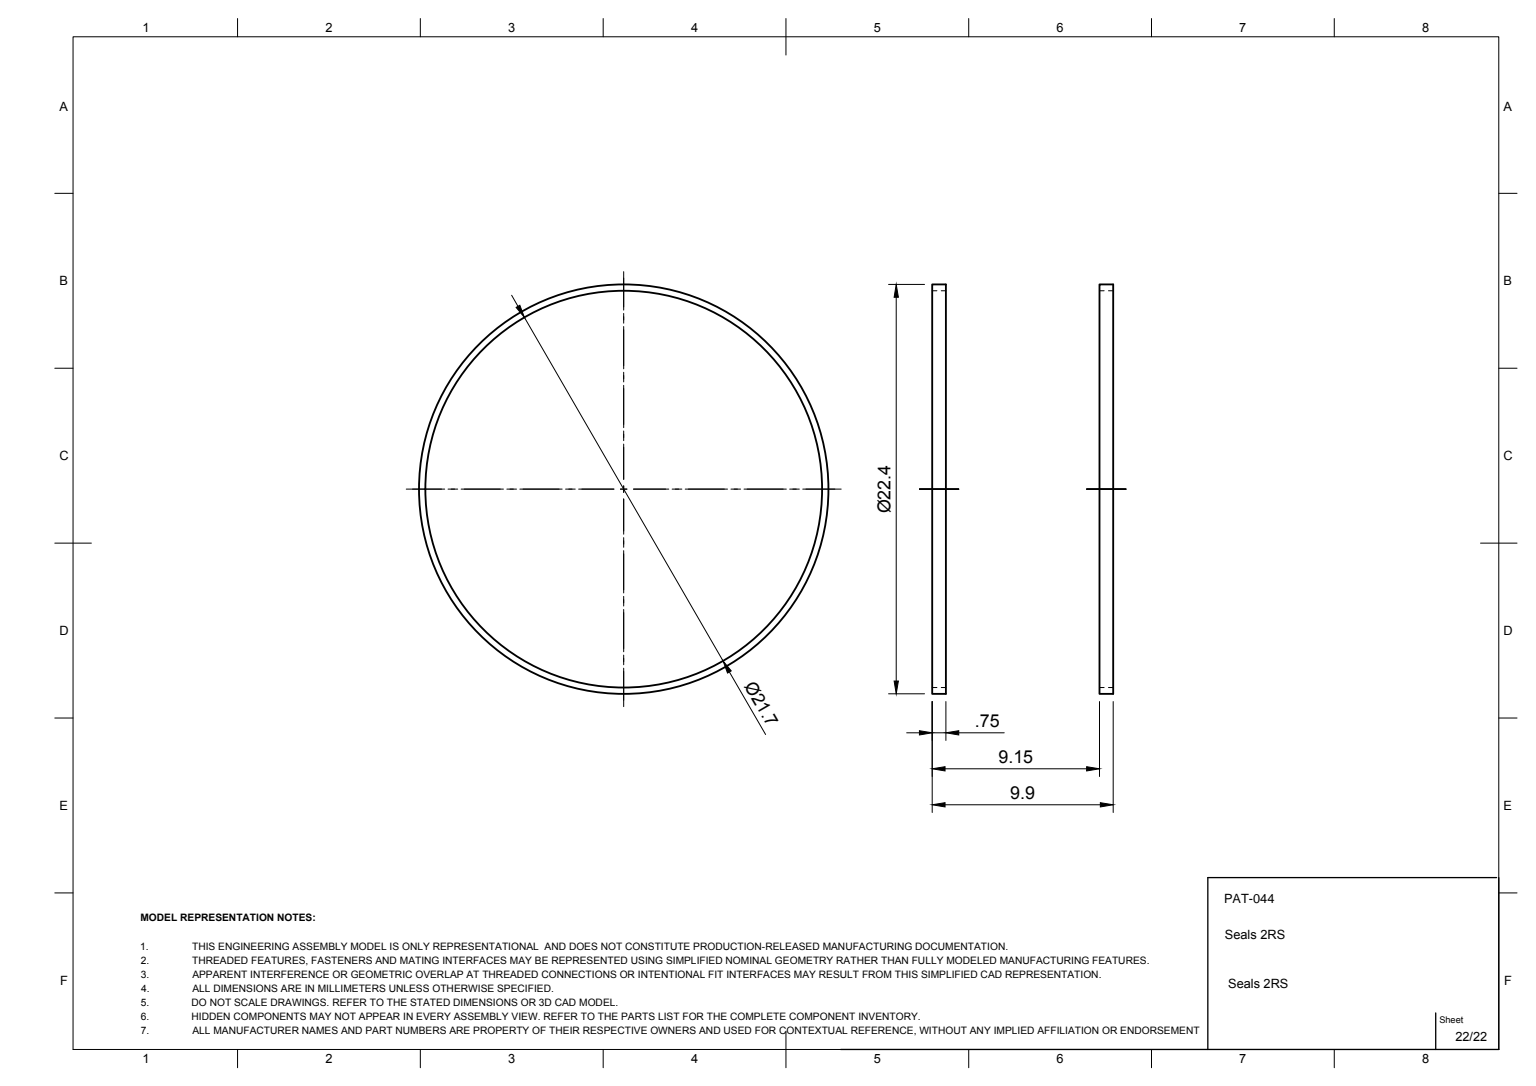
ISO-10303-21;
HEADER;
/* Generated by software containing ST-Developer
 * from STEP Tools, Inc. (www.steptools.com) 
 */

FILE_DESCRIPTION(
/* description */ ('Four-wheel beam trolley'),
/* implementation_level */ '2;1');

FILE_NAME(
/* name */ 'Seals 2RS.step',
/* time_stamp */ '2026-10-29T16:22:06-07:00',
/* author */ (''),
/* organization */ (''),
/* preprocessor_version */ 'ST-DEVELOPER v20.2',
/* originating_system */ 'Autodesk Translation Framework v15.17.0.0',
/* authorisation */ '');

FILE_SCHEMA (('AUTOMOTIVE_DESIGN { 1 0 10303 214 3 1 1 }'));
ENDSEC;

DATA;
#10=MECHANICAL_DESIGN_GEOMETRIC_PRESENTATION_REPRESENTATION('',(#299,#300),#4777);
#259=SHAPE_REPRESENTATION_RELATIONSHIP('SRR','None',#4890,#276);
#276=ADVANCED_BREP_SHAPE_REPRESENTATION('',(#321,#322),#4775);
#299=STYLED_ITEM('',(#5056),#321);
#300=STYLED_ITEM('',(#5056),#322);
#321=MANIFOLD_SOLID_BREP('Body1',#2388);
#322=MANIFOLD_SOLID_BREP('Body2',#2389);
#359=FACE_BOUND('',#760,.T.);
#360=FACE_BOUND('',#763,.T.);
#361=FACE_BOUND('',#766,.T.);
#362=FACE_BOUND('',#769,.T.);
#436=PLANE('',#2892);
#437=PLANE('',#2897);
#438=PLANE('',#2900);
#439=PLANE('',#2905);
#577=FACE_OUTER_BOUND('',#759,.T.);
#578=FACE_OUTER_BOUND('',#761,.T.);
#579=FACE_OUTER_BOUND('',#762,.T.);
#580=FACE_OUTER_BOUND('',#764,.T.);
#581=FACE_OUTER_BOUND('',#765,.T.);
#582=FACE_OUTER_BOUND('',#767,.T.);
#583=FACE_OUTER_BOUND('',#768,.T.);
#584=FACE_OUTER_BOUND('',#770,.T.);
#759=EDGE_LOOP('',(#2139));
#760=EDGE_LOOP('',(#2140));
#761=EDGE_LOOP('',(#2141,#2142,#2143,#2144));
#762=EDGE_LOOP('',(#2145));
#763=EDGE_LOOP('',(#2146));
#764=EDGE_LOOP('',(#2147,#2148,#2149,#2150));
#765=EDGE_LOOP('',(#2151));
#766=EDGE_LOOP('',(#2152));
#767=EDGE_LOOP('',(#2153,#2154,#2155,#2156));
#768=EDGE_LOOP('',(#2157));
#769=EDGE_LOOP('',(#2158));
#770=EDGE_LOOP('',(#2159,#2160,#2161,#2162));
#894=LINE('',#4684,#1017);
#895=LINE('',#4689,#1018);
#896=LINE('',#4698,#1019);
#897=LINE('',#4703,#1020);
#1017=VECTOR('',#3685,1.119765);
#1018=VECTOR('',#3692,1.085235);
#1019=VECTOR('',#3703,1.119765);
#1020=VECTOR('',#3710,1.085235);
#1149=CIRCLE('',#2893,1.119765);
#1150=CIRCLE('',#2894,1.085235);
#1151=CIRCLE('',#2896,1.119765);
#1152=CIRCLE('',#2898,1.085235);
#1153=CIRCLE('',#2901,1.119765);
#1154=CIRCLE('',#2902,1.085235);
#1155=CIRCLE('',#2904,1.119765);
#1156=CIRCLE('',#2906,1.085235);
#1338=VERTEX_POINT('',#4677);
#1339=VERTEX_POINT('',#4679);
#1340=VERTEX_POINT('',#4682);
#1341=VERTEX_POINT('',#4686);
#1342=VERTEX_POINT('',#4691);
#1343=VERTEX_POINT('',#4693);
#1344=VERTEX_POINT('',#4696);
#1345=VERTEX_POINT('',#4700);
#1607=EDGE_CURVE('',#1338,#1338,#1149,.T.);
#1608=EDGE_CURVE('',#1339,#1339,#1150,.T.);
#1609=EDGE_CURVE('',#1340,#1340,#1151,.T.);
#1610=EDGE_CURVE('',#1340,#1338,#894,.T.);
#1611=EDGE_CURVE('',#1341,#1341,#1152,.T.);
#1612=EDGE_CURVE('',#1341,#1339,#895,.T.);
#1613=EDGE_CURVE('',#1342,#1342,#1153,.T.);
#1614=EDGE_CURVE('',#1343,#1343,#1154,.T.);
#1615=EDGE_CURVE('',#1344,#1344,#1155,.T.);
#1616=EDGE_CURVE('',#1344,#1342,#896,.T.);
#1617=EDGE_CURVE('',#1345,#1345,#1156,.T.);
#1618=EDGE_CURVE('',#1345,#1343,#897,.T.);
#2139=ORIENTED_EDGE('',*,*,#1607,.F.);
#2140=ORIENTED_EDGE('',*,*,#1608,.T.);
#2141=ORIENTED_EDGE('',*,*,#1609,.F.);
#2142=ORIENTED_EDGE('',*,*,#1610,.T.);
#2143=ORIENTED_EDGE('',*,*,#1607,.T.);
#2144=ORIENTED_EDGE('',*,*,#1610,.F.);
#2145=ORIENTED_EDGE('',*,*,#1609,.T.);
#2146=ORIENTED_EDGE('',*,*,#1611,.F.);
#2147=ORIENTED_EDGE('',*,*,#1611,.T.);
#2148=ORIENTED_EDGE('',*,*,#1612,.T.);
#2149=ORIENTED_EDGE('',*,*,#1608,.F.);
#2150=ORIENTED_EDGE('',*,*,#1612,.F.);
#2151=ORIENTED_EDGE('',*,*,#1613,.F.);
#2152=ORIENTED_EDGE('',*,*,#1614,.T.);
#2153=ORIENTED_EDGE('',*,*,#1615,.F.);
#2154=ORIENTED_EDGE('',*,*,#1616,.T.);
#2155=ORIENTED_EDGE('',*,*,#1613,.T.);
#2156=ORIENTED_EDGE('',*,*,#1616,.F.);
#2157=ORIENTED_EDGE('',*,*,#1615,.T.);
#2158=ORIENTED_EDGE('',*,*,#1617,.F.);
#2159=ORIENTED_EDGE('',*,*,#1617,.T.);
#2160=ORIENTED_EDGE('',*,*,#1618,.T.);
#2161=ORIENTED_EDGE('',*,*,#1614,.F.);
#2162=ORIENTED_EDGE('',*,*,#1618,.F.);
#2212=CYLINDRICAL_SURFACE('',#2895,1.119765);
#2213=CYLINDRICAL_SURFACE('',#2899,1.085235);
#2214=CYLINDRICAL_SURFACE('',#2903,1.119765);
#2215=CYLINDRICAL_SURFACE('',#2907,1.085235);
#2353=ADVANCED_FACE('',(#577,#359),#436,.T.);
#2354=ADVANCED_FACE('',(#578),#2212,.T.);
#2355=ADVANCED_FACE('',(#579,#360),#437,.T.);
#2356=ADVANCED_FACE('',(#580),#2213,.F.);
#2357=ADVANCED_FACE('',(#581,#361),#438,.T.);
#2358=ADVANCED_FACE('',(#582),#2214,.T.);
#2359=ADVANCED_FACE('',(#583,#362),#439,.T.);
#2360=ADVANCED_FACE('',(#584),#2215,.F.);
#2388=CLOSED_SHELL('',(#2353,#2354,#2355,#2356));
#2389=CLOSED_SHELL('',(#2357,#2358,#2359,#2360));
#2891=AXIS2_PLACEMENT_3D('',#4675,#3673,#3674);
#2892=AXIS2_PLACEMENT_3D('',#4676,#3675,#3676);
#2893=AXIS2_PLACEMENT_3D('',#4678,#3677,#3678);
#2894=AXIS2_PLACEMENT_3D('',#4680,#3679,#3680);
#2895=AXIS2_PLACEMENT_3D('',#4681,#3681,#3682);
#2896=AXIS2_PLACEMENT_3D('',#4683,#3683,#3684);
#2897=AXIS2_PLACEMENT_3D('',#4685,#3686,#3687);
#2898=AXIS2_PLACEMENT_3D('',#4687,#3688,#3689);
#2899=AXIS2_PLACEMENT_3D('',#4688,#3690,#3691);
#2900=AXIS2_PLACEMENT_3D('',#4690,#3693,#3694);
#2901=AXIS2_PLACEMENT_3D('',#4692,#3695,#3696);
#2902=AXIS2_PLACEMENT_3D('',#4694,#3697,#3698);
#2903=AXIS2_PLACEMENT_3D('',#4695,#3699,#3700);
#2904=AXIS2_PLACEMENT_3D('',#4697,#3701,#3702);
#2905=AXIS2_PLACEMENT_3D('',#4699,#3704,#3705);
#2906=AXIS2_PLACEMENT_3D('',#4701,#3706,#3707);
#2907=AXIS2_PLACEMENT_3D('',#4702,#3708,#3709);
#3673=DIRECTION('axis',(0.,0.,1.));
#3674=DIRECTION('refdir',(1.,0.,0.));
#3675=DIRECTION('center_axis',(0.,1.,0.));
#3676=DIRECTION('ref_axis',(0.,0.,1.));
#3677=DIRECTION('center_axis',(0.,-1.,0.));
#3678=DIRECTION('ref_axis',(1.,0.,0.));
#3679=DIRECTION('center_axis',(0.,-1.,0.));
#3680=DIRECTION('ref_axis',(1.,0.,0.));
#3681=DIRECTION('center_axis',(0.,-1.,0.));
#3682=DIRECTION('ref_axis',(1.,0.,0.));
#3683=DIRECTION('center_axis',(0.,-1.,0.));
#3684=DIRECTION('ref_axis',(1.,0.,0.));
#3685=DIRECTION('',(0.,1.,0.));
#3686=DIRECTION('center_axis',(0.,-1.,0.));
#3687=DIRECTION('ref_axis',(0.,0.,-1.));
#3688=DIRECTION('center_axis',(0.,-1.,0.));
#3689=DIRECTION('ref_axis',(1.,0.,0.));
#3690=DIRECTION('center_axis',(0.,-1.,0.));
#3691=DIRECTION('ref_axis',(1.,0.,0.));
#3692=DIRECTION('',(0.,1.,0.));
#3693=DIRECTION('center_axis',(0.,1.,0.));
#3694=DIRECTION('ref_axis',(0.,0.,1.));
#3695=DIRECTION('center_axis',(0.,-1.,0.));
#3696=DIRECTION('ref_axis',(1.,0.,0.));
#3697=DIRECTION('center_axis',(0.,-1.,0.));
#3698=DIRECTION('ref_axis',(1.,0.,0.));
#3699=DIRECTION('center_axis',(0.,-1.,0.));
#3700=DIRECTION('ref_axis',(1.,0.,0.));
#3701=DIRECTION('center_axis',(0.,-1.,0.));
#3702=DIRECTION('ref_axis',(1.,0.,0.));
#3703=DIRECTION('',(0.,1.,0.));
#3704=DIRECTION('center_axis',(0.,-1.,0.));
#3705=DIRECTION('ref_axis',(0.,0.,-1.));
#3706=DIRECTION('center_axis',(0.,-1.,0.));
#3707=DIRECTION('ref_axis',(1.,0.,0.));
#3708=DIRECTION('center_axis',(0.,-1.,0.));
#3709=DIRECTION('ref_axis',(1.,0.,0.));
#3710=DIRECTION('',(0.,1.,0.));
#4675=CARTESIAN_POINT('',(0.,0.,0.));
#4676=CARTESIAN_POINT('Origin',(1.119765,0.495,0.));
#4677=CARTESIAN_POINT('',(-1.119765,0.495,-1.37131662304724E-16));
#4678=CARTESIAN_POINT('Origin',(0.,0.495,0.));
#4679=CARTESIAN_POINT('',(-1.085235,0.495,-1.32902956907268E-16));
#4680=CARTESIAN_POINT('Origin',(0.,0.495,0.));
#4681=CARTESIAN_POINT('Origin',(0.,0.4575,0.));
#4682=CARTESIAN_POINT('',(-1.119765,0.42,-1.37131662304724E-16));
#4683=CARTESIAN_POINT('Origin',(0.,0.42,0.));
#4684=CARTESIAN_POINT('',(-1.119765,0.4575,-1.37131662304724E-16));
#4685=CARTESIAN_POINT('Origin',(1.085235,0.42,0.));
#4686=CARTESIAN_POINT('',(-1.085235,0.42,-1.32902956907268E-16));
#4687=CARTESIAN_POINT('Origin',(0.,0.42,0.));
#4688=CARTESIAN_POINT('Origin',(0.,0.4575,0.));
#4689=CARTESIAN_POINT('',(-1.085235,0.4575,-1.32902956907268E-16));
#4690=CARTESIAN_POINT('Origin',(1.119765,-0.42,0.));
#4691=CARTESIAN_POINT('',(-1.119765,-0.42,-1.37131662304724E-16));
#4692=CARTESIAN_POINT('Origin',(0.,-0.42,0.));
#4693=CARTESIAN_POINT('',(-1.085235,-0.42,-1.32902956907268E-16));
#4694=CARTESIAN_POINT('Origin',(0.,-0.42,0.));
#4695=CARTESIAN_POINT('Origin',(0.,-0.4575,0.));
#4696=CARTESIAN_POINT('',(-1.119765,-0.495,-1.37131662304724E-16));
#4697=CARTESIAN_POINT('Origin',(0.,-0.495,0.));
#4698=CARTESIAN_POINT('',(-1.119765,-0.4575,-1.37131662304724E-16));
#4699=CARTESIAN_POINT('Origin',(1.085235,-0.495,0.));
#4700=CARTESIAN_POINT('',(-1.085235,-0.495,-1.32902956907268E-16));
#4701=CARTESIAN_POINT('Origin',(0.,-0.495,0.));
#4702=CARTESIAN_POINT('Origin',(0.,-0.4575,0.));
#4703=CARTESIAN_POINT('',(-1.085235,-0.4575,-1.32902956907268E-16));
#4753=UNCERTAINTY_MEASURE_WITH_UNIT(LENGTH_MEASURE(0.001),#4778,
'DISTANCE_ACCURACY_VALUE',
'Maximum model space distance between geometric entities at asserted c
onnectivities');
#4755=UNCERTAINTY_MEASURE_WITH_UNIT(LENGTH_MEASURE(0.001),#4778,
'DISTANCE_ACCURACY_VALUE',
'Maximum model space distance between geometric entities at asserted c
onnectivities');
#4775=(
GEOMETRIC_REPRESENTATION_CONTEXT(3)
GLOBAL_UNCERTAINTY_ASSIGNED_CONTEXT((#4753))
GLOBAL_UNIT_ASSIGNED_CONTEXT((#4778,#4780,#4781))
REPRESENTATION_CONTEXT('','3D')
);
#4777=(
GEOMETRIC_REPRESENTATION_CONTEXT(3)
GLOBAL_UNCERTAINTY_ASSIGNED_CONTEXT((#4755))
GLOBAL_UNIT_ASSIGNED_CONTEXT((#4778,#4780,#4781))
REPRESENTATION_CONTEXT('','3D')
);
#4778=(
LENGTH_UNIT()
NAMED_UNIT(*)
SI_UNIT(.CENTI.,.METRE.)
);
#4780=(
NAMED_UNIT(*)
PLANE_ANGLE_UNIT()
SI_UNIT($,.RADIAN.)
);
#4781=(
NAMED_UNIT(*)
SI_UNIT($,.STERADIAN.)
SOLID_ANGLE_UNIT()
);
#4801=SHAPE_DEFINITION_REPRESENTATION(#4854,#4890);
#4854=PRODUCT_DEFINITION_SHAPE('',$,#4912);
#4890=SHAPE_REPRESENTATION('',(#2891),#4775);
#4892=PRODUCT_DEFINITION_CONTEXT('part definition',#4957,'design');
#4912=PRODUCT_DEFINITION('Seals 2RS','Seals 2RS',#4933,#4892);
#4933=PRODUCT_DEFINITION_FORMATION('',$,#4978);
#4957=APPLICATION_CONTEXT(
'Core Data for Automotive Mechanical Design Process');
#4958=PRODUCT_CONTEXT('part definition',#4957,'mechanical');
#4978=PRODUCT('Seals 2RS','Seals 2RS','Seals 2RS',(#4958));
#5050=COLOUR_RGB('Grey',0.48,0.52,0.57);
#5051=FILL_AREA_STYLE_COLOUR('',#5050);
#5052=FILL_AREA_STYLE('',(#5051));
#5053=SURFACE_STYLE_FILL_AREA(#5052);
#5054=SURFACE_SIDE_STYLE('',(#5053));
#5055=SURFACE_STYLE_USAGE(.BOTH.,#5054);
#5056=PRESENTATION_STYLE_ASSIGNMENT((#5055));
ENDSEC;
END-ISO-10303-21;
